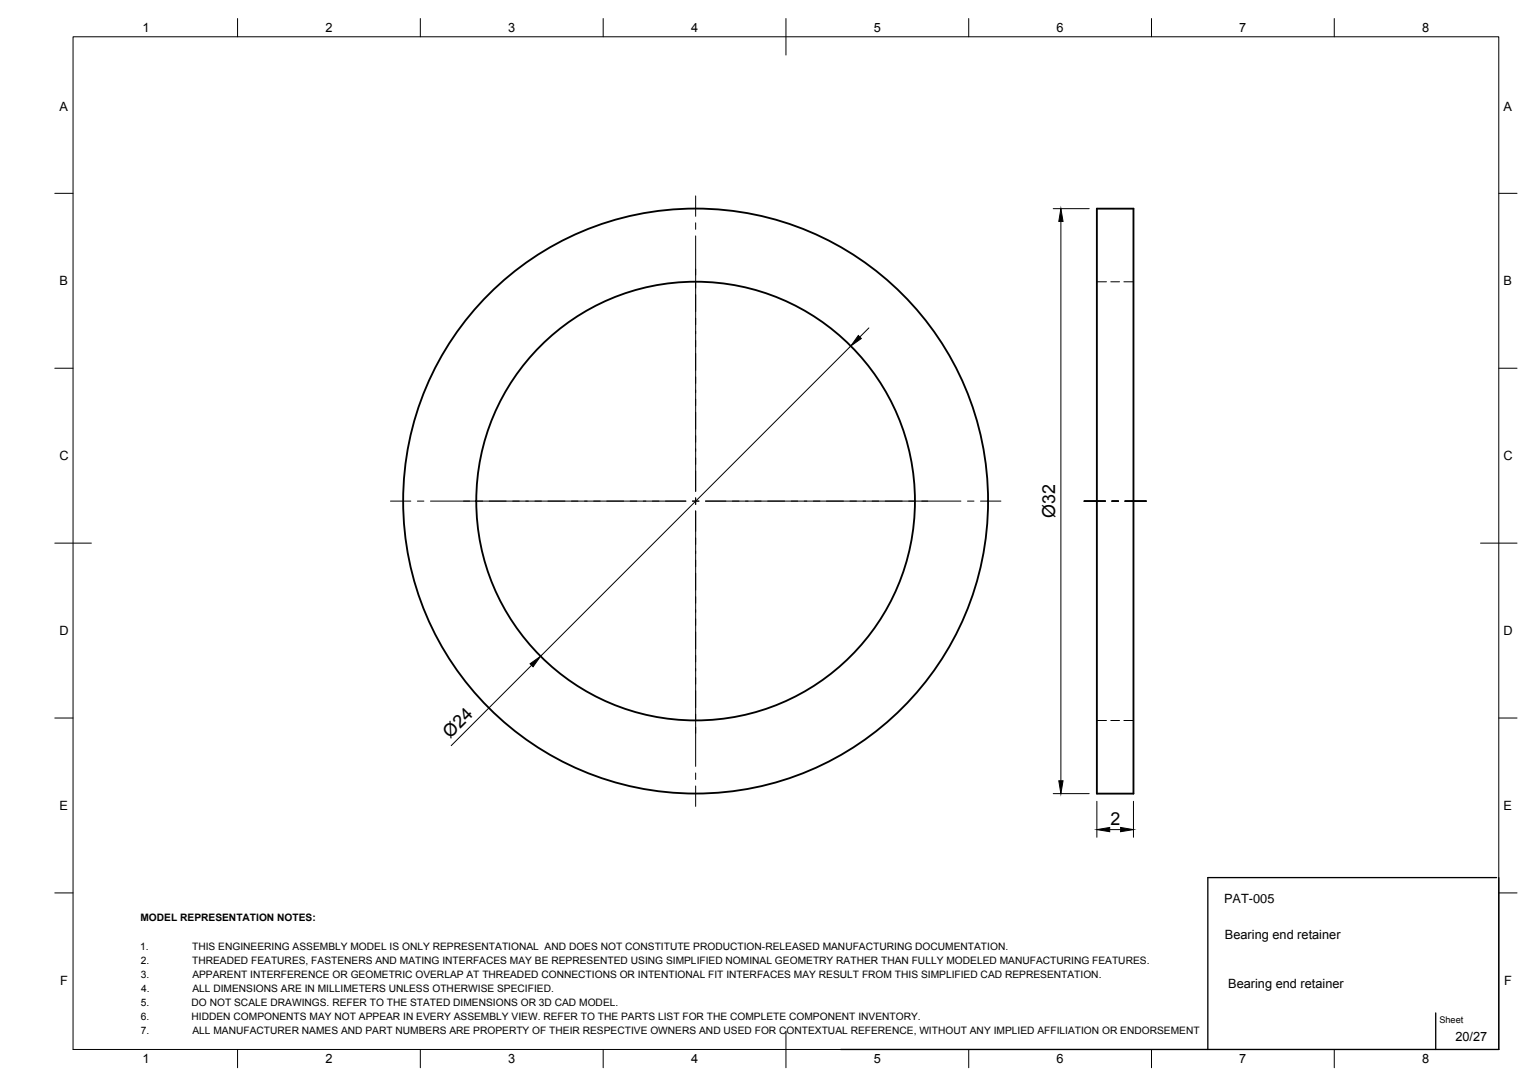
ISO-10303-21;
HEADER;
/* Generated by software containing ST-Developer
 * from STEP Tools, Inc. (www.steptools.com) 
 */

FILE_DESCRIPTION(
/* description */ ('Ball-race swivel caster'),
/* implementation_level */ '2;1');

FILE_NAME(
/* name */ 'Bearing end retainer.step',
/* time_stamp */ '2026-10-29T16:15:51-07:00',
/* author */ (''),
/* organization */ (''),
/* preprocessor_version */ 'ST-DEVELOPER v20.2',
/* originating_system */ 'Autodesk Translation Framework v15.17.0.0',
/* authorisation */ '');

FILE_SCHEMA (('AUTOMOTIVE_DESIGN { 1 0 10303 214 3 1 1 }'));
ENDSEC;

DATA;
#10=MECHANICAL_DESIGN_GEOMETRIC_PRESENTATION_REPRESENTATION('',(#333),#7816);
#277=SHAPE_REPRESENTATION_RELATIONSHIP('SRR','None',#7926,#297);
#297=ADVANCED_BREP_SHAPE_REPRESENTATION('',(#368),#7815);
#333=STYLED_ITEM('',(#8097),#368);
#368=MANIFOLD_SOLID_BREP('Body1',#3740);
#436=FACE_BOUND('',#1008,.T.);
#437=FACE_BOUND('',#1010,.T.);
#522=PLANE('',#4479);
#523=PLANE('',#4480);
#729=FACE_OUTER_BOUND('',#1005,.T.);
#730=FACE_OUTER_BOUND('',#1006,.T.);
#731=FACE_OUTER_BOUND('',#1007,.T.);
#732=FACE_OUTER_BOUND('',#1009,.T.);
#1005=EDGE_LOOP('',(#3415,#3416,#3417,#3418));
#1006=EDGE_LOOP('',(#3419,#3420,#3421,#3422));
#1007=EDGE_LOOP('',(#3423));
#1008=EDGE_LOOP('',(#3424));
#1009=EDGE_LOOP('',(#3425));
#1010=EDGE_LOOP('',(#3426));
#1164=LINE('',#7745,#1319);
#1165=LINE('',#7751,#1320);
#1319=VECTOR('',#5668,1.2);
#1320=VECTOR('',#5675,1.6);
#1581=CIRCLE('',#4474,1.2);
#1582=CIRCLE('',#4475,1.2);
#1583=CIRCLE('',#4477,1.6);
#1584=CIRCLE('',#4478,1.6);
#1932=VERTEX_POINT('',#7742);
#1933=VERTEX_POINT('',#7744);
#1934=VERTEX_POINT('',#7748);
#1935=VERTEX_POINT('',#7750);
#2427=EDGE_CURVE('',#1932,#1932,#1581,.T.);
#2428=EDGE_CURVE('',#1932,#1933,#1164,.T.);
#2429=EDGE_CURVE('',#1933,#1933,#1582,.T.);
#2430=EDGE_CURVE('',#1934,#1934,#1583,.T.);
#2431=EDGE_CURVE('',#1934,#1935,#1165,.T.);
#2432=EDGE_CURVE('',#1935,#1935,#1584,.T.);
#3415=ORIENTED_EDGE('',*,*,#2427,.F.);
#3416=ORIENTED_EDGE('',*,*,#2428,.T.);
#3417=ORIENTED_EDGE('',*,*,#2429,.T.);
#3418=ORIENTED_EDGE('',*,*,#2428,.F.);
#3419=ORIENTED_EDGE('',*,*,#2430,.F.);
#3420=ORIENTED_EDGE('',*,*,#2431,.T.);
#3421=ORIENTED_EDGE('',*,*,#2432,.T.);
#3422=ORIENTED_EDGE('',*,*,#2431,.F.);
#3423=ORIENTED_EDGE('',*,*,#2430,.T.);
#3424=ORIENTED_EDGE('',*,*,#2427,.T.);
#3425=ORIENTED_EDGE('',*,*,#2432,.F.);
#3426=ORIENTED_EDGE('',*,*,#2429,.F.);
#3493=CYLINDRICAL_SURFACE('',#4473,1.2);
#3494=CYLINDRICAL_SURFACE('',#4476,1.6);
#3700=ADVANCED_FACE('',(#729),#3493,.F.);
#3701=ADVANCED_FACE('',(#730),#3494,.T.);
#3702=ADVANCED_FACE('',(#731,#436),#522,.T.);
#3703=ADVANCED_FACE('',(#732,#437),#523,.F.);
#3740=CLOSED_SHELL('',(#3700,#3701,#3702,#3703));
#4472=AXIS2_PLACEMENT_3D('',#7740,#5662,#5663);
#4473=AXIS2_PLACEMENT_3D('',#7741,#5664,#5665);
#4474=AXIS2_PLACEMENT_3D('',#7743,#5666,#5667);
#4475=AXIS2_PLACEMENT_3D('',#7746,#5669,#5670);
#4476=AXIS2_PLACEMENT_3D('',#7747,#5671,#5672);
#4477=AXIS2_PLACEMENT_3D('',#7749,#5673,#5674);
#4478=AXIS2_PLACEMENT_3D('',#7752,#5676,#5677);
#4479=AXIS2_PLACEMENT_3D('',#7753,#5678,#5679);
#4480=AXIS2_PLACEMENT_3D('',#7754,#5680,#5681);
#5662=DIRECTION('axis',(0.,0.,1.));
#5663=DIRECTION('refdir',(1.,0.,0.));
#5664=DIRECTION('center_axis',(0.,1.,0.));
#5665=DIRECTION('ref_axis',(1.,0.,0.));
#5666=DIRECTION('center_axis',(0.,-1.,0.));
#5667=DIRECTION('ref_axis',(1.,0.,0.));
#5668=DIRECTION('',(0.,-1.,0.));
#5669=DIRECTION('center_axis',(0.,-1.,0.));
#5670=DIRECTION('ref_axis',(1.,0.,0.));
#5671=DIRECTION('center_axis',(0.,1.,0.));
#5672=DIRECTION('ref_axis',(1.,0.,0.));
#5673=DIRECTION('center_axis',(0.,1.,0.));
#5674=DIRECTION('ref_axis',(1.,0.,0.));
#5675=DIRECTION('',(0.,-1.,0.));
#5676=DIRECTION('center_axis',(0.,1.,0.));
#5677=DIRECTION('ref_axis',(1.,0.,0.));
#5678=DIRECTION('center_axis',(0.,1.,0.));
#5679=DIRECTION('ref_axis',(1.,0.,0.));
#5680=DIRECTION('center_axis',(0.,1.,0.));
#5681=DIRECTION('ref_axis',(1.,0.,0.));
#7740=CARTESIAN_POINT('',(0.,0.,0.));
#7741=CARTESIAN_POINT('Origin',(0.,1.1,3.5));
#7742=CARTESIAN_POINT('',(-1.2,1.3,3.5));
#7743=CARTESIAN_POINT('Origin',(0.,1.3,3.5));
#7744=CARTESIAN_POINT('',(-1.2,1.1,3.5));
#7745=CARTESIAN_POINT('',(-1.2,1.1,3.5));
#7746=CARTESIAN_POINT('Origin',(0.,1.1,3.5));
#7747=CARTESIAN_POINT('Origin',(0.,1.1,3.5));
#7748=CARTESIAN_POINT('',(-1.6,1.3,3.5));
#7749=CARTESIAN_POINT('Origin',(0.,1.3,3.5));
#7750=CARTESIAN_POINT('',(-1.6,1.1,3.5));
#7751=CARTESIAN_POINT('',(-1.6,1.1,3.5));
#7752=CARTESIAN_POINT('Origin',(0.,1.1,3.5));
#7753=CARTESIAN_POINT('Origin',(0.,1.3,3.5));
#7754=CARTESIAN_POINT('Origin',(0.,1.1,3.5));
#7788=UNCERTAINTY_MEASURE_WITH_UNIT(LENGTH_MEASURE(0.001),#7817,
'DISTANCE_ACCURACY_VALUE',
'Maximum model space distance between geometric entities at asserted c
onnectivities');
#7789=UNCERTAINTY_MEASURE_WITH_UNIT(LENGTH_MEASURE(0.001),#7817,
'DISTANCE_ACCURACY_VALUE',
'Maximum model space distance between geometric entities at asserted c
onnectivities');
#7815=(
GEOMETRIC_REPRESENTATION_CONTEXT(3)
GLOBAL_UNCERTAINTY_ASSIGNED_CONTEXT((#7788))
GLOBAL_UNIT_ASSIGNED_CONTEXT((#7817,#7819,#7820))
REPRESENTATION_CONTEXT('','3D')
);
#7816=(
GEOMETRIC_REPRESENTATION_CONTEXT(3)
GLOBAL_UNCERTAINTY_ASSIGNED_CONTEXT((#7789))
GLOBAL_UNIT_ASSIGNED_CONTEXT((#7817,#7819,#7820))
REPRESENTATION_CONTEXT('','3D')
);
#7817=(
LENGTH_UNIT()
NAMED_UNIT(*)
SI_UNIT(.CENTI.,.METRE.)
);
#7819=(
NAMED_UNIT(*)
PLANE_ANGLE_UNIT()
SI_UNIT($,.RADIAN.)
);
#7820=(
NAMED_UNIT(*)
SI_UNIT($,.STERADIAN.)
SOLID_ANGLE_UNIT()
);
#7846=SHAPE_DEFINITION_REPRESENTATION(#7892,#7926);
#7892=PRODUCT_DEFINITION_SHAPE('',$,#7953);
#7926=SHAPE_REPRESENTATION('',(#4472),#7815);
#7927=PRODUCT_DEFINITION_CONTEXT('part definition',#8007,'design');
#7953=PRODUCT_DEFINITION('Bearing end retainer','Bearing end retainer',
#7979,#7927);
#7979=PRODUCT_DEFINITION_FORMATION('',$,#8034);
#8007=APPLICATION_CONTEXT(
'Core Data for Automotive Mechanical Design Process');
#8008=PRODUCT_CONTEXT('part definition',#8007,'mechanical');
#8034=PRODUCT('Bearing end retainer','Bearing end retainer',
'Bearing end retainer',(#8008));
#8091=COLOUR_RGB('Grey',0.48,0.52,0.57);
#8092=FILL_AREA_STYLE_COLOUR('',#8091);
#8093=FILL_AREA_STYLE('',(#8092));
#8094=SURFACE_STYLE_FILL_AREA(#8093);
#8095=SURFACE_SIDE_STYLE('',(#8094));
#8096=SURFACE_STYLE_USAGE(.BOTH.,#8095);
#8097=PRESENTATION_STYLE_ASSIGNMENT((#8096));
ENDSEC;
END-ISO-10303-21;
